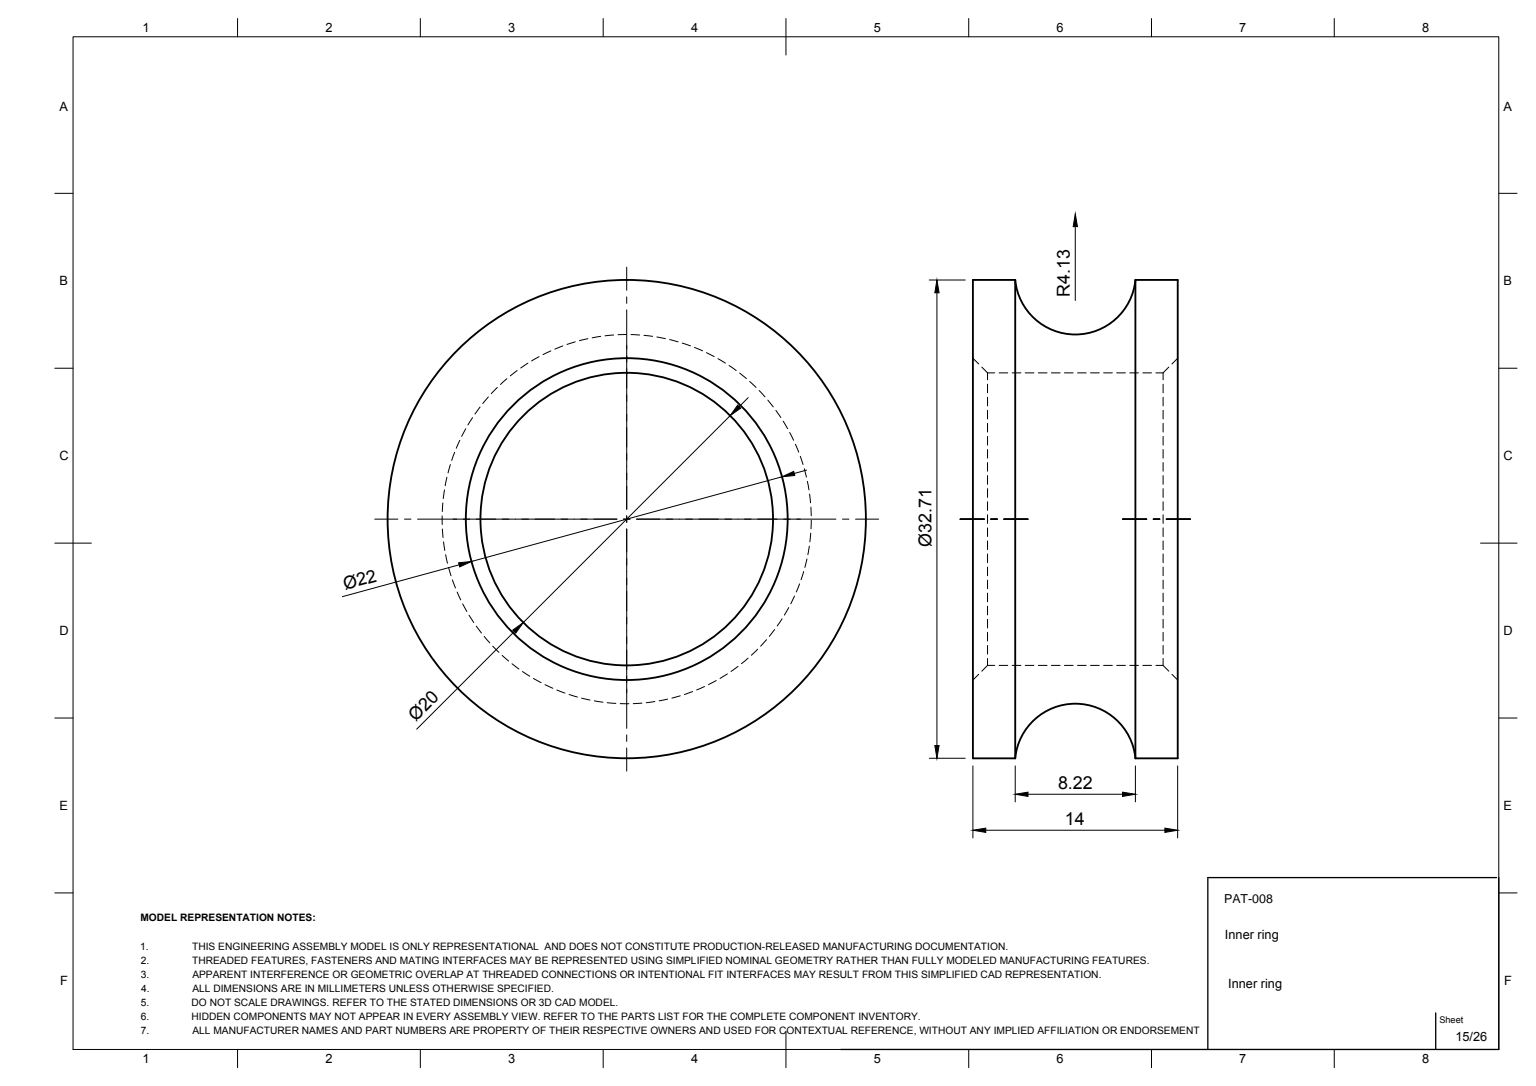
ISO-10303-21;
HEADER;
/* Generated by software containing ST-Developer
 * from STEP Tools, Inc. (www.steptools.com) 
 */

FILE_DESCRIPTION(
/* description */ ('Bearing housing with oil seal and end cap'),
/* implementation_level */ '2;1');

FILE_NAME(
/* name */ 'Inner ring.step',
/* time_stamp */ '2026-10-28T03:23:10-07:00',
/* author */ (''),
/* organization */ (''),
/* preprocessor_version */ 'ST-DEVELOPER v20.2',
/* originating_system */ 'Autodesk Translation Framework v15.17.0.0',
/* authorisation */ '');

FILE_SCHEMA (('AUTOMOTIVE_DESIGN { 1 0 10303 214 3 1 1 }'));
ENDSEC;

DATA;
#10=MECHANICAL_DESIGN_GEOMETRIC_PRESENTATION_REPRESENTATION('',(#267),#7871);
#201=CONICAL_SURFACE('',#4568,1.05,0.785398163397449);
#202=CONICAL_SURFACE('',#4575,1.05,0.785398163397449);
#215=TOROIDAL_SURFACE('',#4557,1.675,0.412776);
#225=SHAPE_REPRESENTATION_RELATIONSHIP('SRR','None',#7973,#246);
#246=ADVANCED_BREP_SHAPE_REPRESENTATION('',(#296),#7857);
#267=STYLED_ITEM('',(#8153),#296);
#296=MANIFOLD_SOLID_BREP('Body1',#4093);
#374=FACE_BOUND('',#972,.T.);
#375=FACE_BOUND('',#975,.T.);
#471=PLANE('',#4570);
#472=PLANE('',#4573);
#657=FACE_OUTER_BOUND('',#967,.T.);
#658=FACE_OUTER_BOUND('',#968,.T.);
#659=FACE_OUTER_BOUND('',#969,.T.);
#660=FACE_OUTER_BOUND('',#970,.T.);
#661=FACE_OUTER_BOUND('',#971,.T.);
#662=FACE_OUTER_BOUND('',#973,.T.);
#663=FACE_OUTER_BOUND('',#974,.T.);
#664=FACE_OUTER_BOUND('',#976,.T.);
#967=EDGE_LOOP('',(#3155,#3156,#3157,#3158,#3159,#3160));
#968=EDGE_LOOP('',(#3161,#3162,#3163,#3164,#3165));
#969=EDGE_LOOP('',(#3166,#3167,#3168,#3169));
#970=EDGE_LOOP('',(#3170,#3171,#3172,#3173));
#971=EDGE_LOOP('',(#3174));
#972=EDGE_LOOP('',(#3175));
#973=EDGE_LOOP('',(#3176,#3177,#3178,#3179,#3180));
#974=EDGE_LOOP('',(#3181));
#975=EDGE_LOOP('',(#3182));
#976=EDGE_LOOP('',(#3183,#3184,#3185,#3186));
#1261=LINE('',#6677,#1523);
#1262=LINE('',#6683,#1524);
#1263=LINE('',#6687,#1525);
#1264=LINE('',#6693,#1526);
#1265=LINE('',#6698,#1527);
#1523=VECTOR('',#5426,1.63531);
#1524=VECTOR('',#5433,1.);
#1525=VECTOR('',#5438,1.05);
#1526=VECTOR('',#5447,1.63531);
#1527=VECTOR('',#5454,1.05);
#1763=CIRCLE('',#4558,1.63531);
#1764=CIRCLE('',#4559,1.63531);
#1765=CIRCLE('',#4560,0.412776);
#1766=CIRCLE('',#4561,1.63531);
#1767=CIRCLE('',#4562,1.63531);
#1768=CIRCLE('',#4564,1.63531);
#1769=CIRCLE('',#4566,1.);
#1770=CIRCLE('',#4567,1.);
#1771=CIRCLE('',#4569,1.1);
#1772=CIRCLE('',#4572,1.63531);
#1773=CIRCLE('',#4574,1.1);
#2027=VERTEX_POINT('',#6666);
#2028=VERTEX_POINT('',#6667);
#2029=VERTEX_POINT('',#6670);
#2030=VERTEX_POINT('',#6672);
#2031=VERTEX_POINT('',#6676);
#2032=VERTEX_POINT('',#6680);
#2033=VERTEX_POINT('',#6682);
#2034=VERTEX_POINT('',#6686);
#2035=VERTEX_POINT('',#6691);
#2036=VERTEX_POINT('',#6695);
#2441=EDGE_CURVE('',#2027,#2028,#1763,.T.);
#2442=EDGE_CURVE('',#2028,#2027,#1764,.T.);
#2443=EDGE_CURVE('',#2028,#2029,#1765,.T.);
#2444=EDGE_CURVE('',#2030,#2029,#1766,.T.);
#2445=EDGE_CURVE('',#2029,#2030,#1767,.T.);
#2446=EDGE_CURVE('',#2030,#2031,#1261,.T.);
#2447=EDGE_CURVE('',#2031,#2031,#1768,.T.);
#2448=EDGE_CURVE('',#2032,#2032,#1769,.T.);
#2449=EDGE_CURVE('',#2032,#2033,#1262,.T.);
#2450=EDGE_CURVE('',#2033,#2033,#1770,.T.);
#2451=EDGE_CURVE('',#2033,#2034,#1263,.T.);
#2452=EDGE_CURVE('',#2034,#2034,#1771,.T.);
#2453=EDGE_CURVE('',#2035,#2035,#1772,.T.);
#2454=EDGE_CURVE('',#2035,#2027,#1264,.T.);
#2455=EDGE_CURVE('',#2036,#2036,#1773,.T.);
#2456=EDGE_CURVE('',#2036,#2032,#1265,.T.);
#3155=ORIENTED_EDGE('',*,*,#2441,.F.);
#3156=ORIENTED_EDGE('',*,*,#2442,.F.);
#3157=ORIENTED_EDGE('',*,*,#2443,.T.);
#3158=ORIENTED_EDGE('',*,*,#2444,.F.);
#3159=ORIENTED_EDGE('',*,*,#2445,.F.);
#3160=ORIENTED_EDGE('',*,*,#2443,.F.);
#3161=ORIENTED_EDGE('',*,*,#2444,.T.);
#3162=ORIENTED_EDGE('',*,*,#2445,.T.);
#3163=ORIENTED_EDGE('',*,*,#2446,.T.);
#3164=ORIENTED_EDGE('',*,*,#2447,.T.);
#3165=ORIENTED_EDGE('',*,*,#2446,.F.);
#3166=ORIENTED_EDGE('',*,*,#2448,.T.);
#3167=ORIENTED_EDGE('',*,*,#2449,.T.);
#3168=ORIENTED_EDGE('',*,*,#2450,.F.);
#3169=ORIENTED_EDGE('',*,*,#2449,.F.);
#3170=ORIENTED_EDGE('',*,*,#2450,.T.);
#3171=ORIENTED_EDGE('',*,*,#2451,.T.);
#3172=ORIENTED_EDGE('',*,*,#2452,.F.);
#3173=ORIENTED_EDGE('',*,*,#2451,.F.);
#3174=ORIENTED_EDGE('',*,*,#2447,.F.);
#3175=ORIENTED_EDGE('',*,*,#2452,.T.);
#3176=ORIENTED_EDGE('',*,*,#2453,.F.);
#3177=ORIENTED_EDGE('',*,*,#2454,.T.);
#3178=ORIENTED_EDGE('',*,*,#2441,.T.);
#3179=ORIENTED_EDGE('',*,*,#2442,.T.);
#3180=ORIENTED_EDGE('',*,*,#2454,.F.);
#3181=ORIENTED_EDGE('',*,*,#2453,.T.);
#3182=ORIENTED_EDGE('',*,*,#2455,.F.);
#3183=ORIENTED_EDGE('',*,*,#2455,.T.);
#3184=ORIENTED_EDGE('',*,*,#2456,.T.);
#3185=ORIENTED_EDGE('',*,*,#2448,.F.);
#3186=ORIENTED_EDGE('',*,*,#2456,.F.);
#3801=CYLINDRICAL_SURFACE('',#4563,1.63531);
#3802=CYLINDRICAL_SURFACE('',#4565,1.);
#3803=CYLINDRICAL_SURFACE('',#4571,1.63531);
#3939=ADVANCED_FACE('',(#657),#215,.F.);
#3940=ADVANCED_FACE('',(#658),#3801,.T.);
#3941=ADVANCED_FACE('',(#659),#3802,.F.);
#3942=ADVANCED_FACE('',(#660),#201,.F.);
#3943=ADVANCED_FACE('',(#661,#374),#471,.T.);
#3944=ADVANCED_FACE('',(#662),#3803,.T.);
#3945=ADVANCED_FACE('',(#663,#375),#472,.T.);
#3946=ADVANCED_FACE('',(#664),#202,.F.);
#4093=CLOSED_SHELL('',(#3939,#3940,#3941,#3942,#3943,#3944,#3945,#3946));
#4556=AXIS2_PLACEMENT_3D('',#6664,#5410,#5411);
#4557=AXIS2_PLACEMENT_3D('',#6665,#5412,#5413);
#4558=AXIS2_PLACEMENT_3D('',#6668,#5414,#5415);
#4559=AXIS2_PLACEMENT_3D('',#6669,#5416,#5417);
#4560=AXIS2_PLACEMENT_3D('',#6671,#5418,#5419);
#4561=AXIS2_PLACEMENT_3D('',#6673,#5420,#5421);
#4562=AXIS2_PLACEMENT_3D('',#6674,#5422,#5423);
#4563=AXIS2_PLACEMENT_3D('',#6675,#5424,#5425);
#4564=AXIS2_PLACEMENT_3D('',#6678,#5427,#5428);
#4565=AXIS2_PLACEMENT_3D('',#6679,#5429,#5430);
#4566=AXIS2_PLACEMENT_3D('',#6681,#5431,#5432);
#4567=AXIS2_PLACEMENT_3D('',#6684,#5434,#5435);
#4568=AXIS2_PLACEMENT_3D('',#6685,#5436,#5437);
#4569=AXIS2_PLACEMENT_3D('',#6688,#5439,#5440);
#4570=AXIS2_PLACEMENT_3D('',#6689,#5441,#5442);
#4571=AXIS2_PLACEMENT_3D('',#6690,#5443,#5444);
#4572=AXIS2_PLACEMENT_3D('',#6692,#5445,#5446);
#4573=AXIS2_PLACEMENT_3D('',#6694,#5448,#5449);
#4574=AXIS2_PLACEMENT_3D('',#6696,#5450,#5451);
#4575=AXIS2_PLACEMENT_3D('',#6697,#5452,#5453);
#5410=DIRECTION('axis',(0.,0.,1.));
#5411=DIRECTION('refdir',(1.,0.,0.));
#5412=DIRECTION('center_axis',(0.,-1.,0.));
#5413=DIRECTION('ref_axis',(0.,0.,-1.));
#5414=DIRECTION('center_axis',(0.,-1.,0.));
#5415=DIRECTION('ref_axis',(1.,0.,0.));
#5416=DIRECTION('center_axis',(0.,-1.,0.));
#5417=DIRECTION('ref_axis',(1.,0.,0.));
#5418=DIRECTION('center_axis',(1.,0.,1.22464679914735E-16));
#5419=DIRECTION('ref_axis',(-1.22464679914735E-16,0.,1.));
#5420=DIRECTION('center_axis',(0.,1.,0.));
#5421=DIRECTION('ref_axis',(1.,0.,0.));
#5422=DIRECTION('center_axis',(0.,1.,0.));
#5423=DIRECTION('ref_axis',(1.,0.,0.));
#5424=DIRECTION('center_axis',(0.,-1.,0.));
#5425=DIRECTION('ref_axis',(1.,0.,0.));
#5426=DIRECTION('',(0.,1.,0.));
#5427=DIRECTION('center_axis',(0.,-1.,0.));
#5428=DIRECTION('ref_axis',(1.,0.,0.));
#5429=DIRECTION('center_axis',(0.,-1.,0.));
#5430=DIRECTION('ref_axis',(1.,0.,0.));
#5431=DIRECTION('center_axis',(0.,-1.,0.));
#5432=DIRECTION('ref_axis',(1.,0.,0.));
#5433=DIRECTION('',(0.,1.,0.));
#5434=DIRECTION('center_axis',(0.,-1.,0.));
#5435=DIRECTION('ref_axis',(1.,0.,0.));
#5436=DIRECTION('center_axis',(0.,1.,0.));
#5437=DIRECTION('ref_axis',(1.,0.,0.));
#5438=DIRECTION('',(-0.707106781186548,0.707106781186547,-8.65956056235494E-17));
#5439=DIRECTION('center_axis',(0.,-1.,0.));
#5440=DIRECTION('ref_axis',(1.,0.,0.));
#5441=DIRECTION('center_axis',(0.,1.,0.));
#5442=DIRECTION('ref_axis',(0.,0.,1.));
#5443=DIRECTION('center_axis',(0.,-1.,0.));
#5444=DIRECTION('ref_axis',(1.,0.,0.));
#5445=DIRECTION('center_axis',(0.,-1.,0.));
#5446=DIRECTION('ref_axis',(1.,0.,0.));
#5447=DIRECTION('',(0.,1.,0.));
#5448=DIRECTION('center_axis',(0.,-1.,0.));
#5449=DIRECTION('ref_axis',(0.,0.,-1.));
#5450=DIRECTION('center_axis',(0.,-1.,0.));
#5451=DIRECTION('ref_axis',(1.,0.,0.));
#5452=DIRECTION('center_axis',(0.,-1.,0.));
#5453=DIRECTION('ref_axis',(1.,0.,0.));
#5454=DIRECTION('',(0.707106781186548,0.707106781186547,8.65956056235494E-17));
#6664=CARTESIAN_POINT('',(0.,0.,0.));
#6665=CARTESIAN_POINT('Origin',(0.,0.,0.));
#6666=CARTESIAN_POINT('',(-1.63531,-0.410863395882378,-2.00267715711366E-16));
#6667=CARTESIAN_POINT('',(-2.00267715711366E-16,-0.410863395882378,1.63531));
#6668=CARTESIAN_POINT('Origin',(0.,-0.410863395882378,0.));
#6669=CARTESIAN_POINT('Origin',(0.,-0.410863395882378,0.));
#6670=CARTESIAN_POINT('',(-2.00267715711366E-16,0.410863395882378,1.63531));
#6671=CARTESIAN_POINT('Origin',(-2.05128338857182E-16,0.,1.675));
#6672=CARTESIAN_POINT('',(-1.63531,0.410863395882378,2.00267715711366E-16));
#6673=CARTESIAN_POINT('Origin',(0.,0.410863395882378,0.));
#6674=CARTESIAN_POINT('Origin',(0.,0.410863395882378,0.));
#6675=CARTESIAN_POINT('Origin',(0.,0.,0.));
#6676=CARTESIAN_POINT('',(-1.63531,0.7,-2.00267715711366E-16));
#6677=CARTESIAN_POINT('',(-1.63531,0.,-2.00267715711366E-16));
#6678=CARTESIAN_POINT('Origin',(0.,0.7,0.));
#6679=CARTESIAN_POINT('Origin',(0.,0.,0.));
#6680=CARTESIAN_POINT('',(-1.,-0.6,-1.22464679914735E-16));
#6681=CARTESIAN_POINT('Origin',(0.,-0.6,0.));
#6682=CARTESIAN_POINT('',(-1.,0.6,-1.22464679914735E-16));
#6683=CARTESIAN_POINT('',(-1.,0.,-1.22464679914735E-16));
#6684=CARTESIAN_POINT('Origin',(0.,0.6,0.));
#6685=CARTESIAN_POINT('Origin',(0.,0.65,0.));
#6686=CARTESIAN_POINT('',(-1.1,0.7,-1.34711147906209E-16));
#6687=CARTESIAN_POINT('',(-1.05,0.65,-1.28587913910472E-16));
#6688=CARTESIAN_POINT('Origin',(0.,0.7,0.));
#6689=CARTESIAN_POINT('Origin',(1.63531,0.7,0.));
#6690=CARTESIAN_POINT('Origin',(0.,0.,0.));
#6691=CARTESIAN_POINT('',(-1.63531,-0.7,-2.00267715711366E-16));
#6692=CARTESIAN_POINT('Origin',(0.,-0.7,0.));
#6693=CARTESIAN_POINT('',(-1.63531,0.,-2.00267715711366E-16));
#6694=CARTESIAN_POINT('Origin',(1.1,-0.7,0.));
#6695=CARTESIAN_POINT('',(-1.1,-0.7,-1.34711147906209E-16));
#6696=CARTESIAN_POINT('Origin',(0.,-0.7,0.));
#6697=CARTESIAN_POINT('Origin',(0.,-0.65,0.));
#6698=CARTESIAN_POINT('',(-1.05,-0.65,-1.28587913910472E-16));
#7831=UNCERTAINTY_MEASURE_WITH_UNIT(LENGTH_MEASURE(0.001),#7872,
'DISTANCE_ACCURACY_VALUE',
'Maximum model space distance between geometric entities at asserted c
onnectivities');
#7845=UNCERTAINTY_MEASURE_WITH_UNIT(LENGTH_MEASURE(0.001),#7872,
'DISTANCE_ACCURACY_VALUE',
'Maximum model space distance between geometric entities at asserted c
onnectivities');
#7857=(
GEOMETRIC_REPRESENTATION_CONTEXT(3)
GLOBAL_UNCERTAINTY_ASSIGNED_CONTEXT((#7831))
GLOBAL_UNIT_ASSIGNED_CONTEXT((#7872,#7874,#7875))
REPRESENTATION_CONTEXT('','3D')
);
#7871=(
GEOMETRIC_REPRESENTATION_CONTEXT(3)
GLOBAL_UNCERTAINTY_ASSIGNED_CONTEXT((#7845))
GLOBAL_UNIT_ASSIGNED_CONTEXT((#7872,#7874,#7875))
REPRESENTATION_CONTEXT('','3D')
);
#7872=(
LENGTH_UNIT()
NAMED_UNIT(*)
SI_UNIT(.CENTI.,.METRE.)
);
#7874=(
NAMED_UNIT(*)
PLANE_ANGLE_UNIT()
SI_UNIT($,.RADIAN.)
);
#7875=(
NAMED_UNIT(*)
SI_UNIT($,.STERADIAN.)
SOLID_ANGLE_UNIT()
);
#7887=SHAPE_DEFINITION_REPRESENTATION(#7912,#7973);
#7912=PRODUCT_DEFINITION_SHAPE('',$,#7999);
#7973=SHAPE_REPRESENTATION('',(#4556),#7857);
#7987=PRODUCT_DEFINITION_CONTEXT('part definition',#8064,'design');
#7999=PRODUCT_DEFINITION('Inner ring','Inner ring',#8024,#7987);
#8024=PRODUCT_DEFINITION_FORMATION('',$,#8077);
#8064=APPLICATION_CONTEXT(
'Core Data for Automotive Mechanical Design Process');
#8065=PRODUCT_CONTEXT('part definition',#8064,'mechanical');
#8077=PRODUCT('Inner ring','Inner ring','Inner ring',(#8065));
#8147=COLOUR_RGB('Grey',0.48,0.52,0.57);
#8148=FILL_AREA_STYLE_COLOUR('',#8147);
#8149=FILL_AREA_STYLE('',(#8148));
#8150=SURFACE_STYLE_FILL_AREA(#8149);
#8151=SURFACE_SIDE_STYLE('',(#8150));
#8152=SURFACE_STYLE_USAGE(.BOTH.,#8151);
#8153=PRESENTATION_STYLE_ASSIGNMENT((#8152));
ENDSEC;
END-ISO-10303-21;
